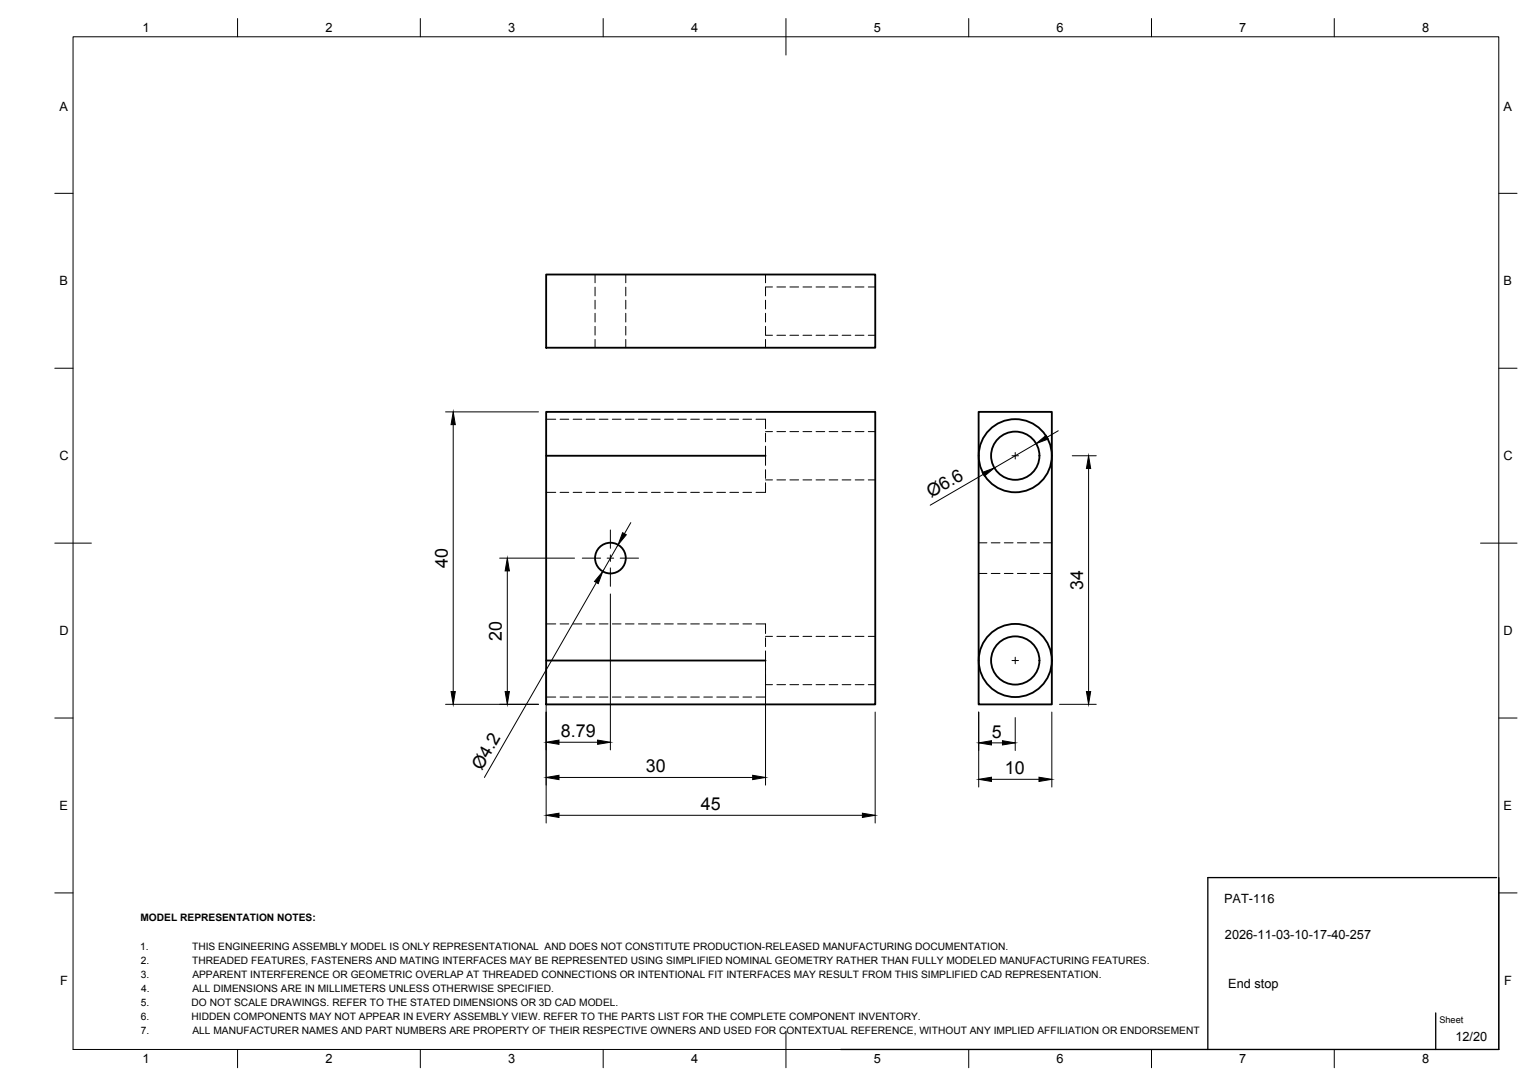
ISO-10303-21;
HEADER;
/* Generated by software containing ST-Developer
 * from STEP Tools, Inc. (www.steptools.com) 
 */

FILE_DESCRIPTION(
/* description */ ('V-block with clamp strap'),
/* implementation_level */ '2;1');

FILE_NAME(
/* name */ 'End stop.step',
/* time_stamp */ '2026-10-27T10:50:53-07:00',
/* author */ (''),
/* organization */ (''),
/* preprocessor_version */ 'ST-DEVELOPER v20.2',
/* originating_system */ 'Autodesk Translation Framework v15.17.0.0',
/* authorisation */ '');

FILE_SCHEMA (('AUTOMOTIVE_DESIGN { 1 0 10303 214 3 1 1 }'));
ENDSEC;

DATA;
#10=MECHANICAL_DESIGN_GEOMETRIC_PRESENTATION_REPRESENTATION('',(#273),#7344);
#231=SHAPE_REPRESENTATION_RELATIONSHIP('SRR','None',#7449,#252);
#252=ADVANCED_BREP_SHAPE_REPRESENTATION('',(#294),#7328);
#273=STYLED_ITEM('',(#7624),#294);
#294=MANIFOLD_SOLID_BREP('Body1',#4155);
#349=FACE_BOUND('',#954,.T.);
#350=FACE_BOUND('',#958,.T.);
#351=FACE_BOUND('',#966,.T.);
#352=FACE_BOUND('',#969,.T.);
#353=FACE_BOUND('',#971,.T.);
#354=FACE_BOUND('',#972,.T.);
#432=CIRCLE('',#4579,0.21);
#433=CIRCLE('',#4580,0.21);
#434=CIRCLE('',#4582,0.5);
#435=CIRCLE('',#4583,0.5);
#436=CIRCLE('',#4585,0.5);
#437=CIRCLE('',#4586,0.5);
#438=CIRCLE('',#4588,0.33);
#439=CIRCLE('',#4590,0.5);
#440=CIRCLE('',#4591,0.5);
#441=CIRCLE('',#4593,0.5);
#442=CIRCLE('',#4594,0.5);
#443=CIRCLE('',#4596,0.33);
#444=CIRCLE('',#4601,0.33);
#445=CIRCLE('',#4603,0.33);
#533=CYLINDRICAL_SURFACE('',#4578,0.21);
#534=CYLINDRICAL_SURFACE('',#4581,0.5);
#535=CYLINDRICAL_SURFACE('',#4584,0.5);
#536=CYLINDRICAL_SURFACE('',#4589,0.5);
#537=CYLINDRICAL_SURFACE('',#4592,0.5);
#538=CYLINDRICAL_SURFACE('',#4600,0.33);
#539=CYLINDRICAL_SURFACE('',#4602,0.33);
#666=FACE_OUTER_BOUND('',#950,.T.);
#667=FACE_OUTER_BOUND('',#951,.T.);
#668=FACE_OUTER_BOUND('',#952,.T.);
#669=FACE_OUTER_BOUND('',#953,.T.);
#670=FACE_OUTER_BOUND('',#955,.T.);
#671=FACE_OUTER_BOUND('',#956,.T.);
#672=FACE_OUTER_BOUND('',#957,.T.);
#673=FACE_OUTER_BOUND('',#959,.T.);
#674=FACE_OUTER_BOUND('',#960,.T.);
#675=FACE_OUTER_BOUND('',#961,.T.);
#676=FACE_OUTER_BOUND('',#962,.T.);
#677=FACE_OUTER_BOUND('',#963,.T.);
#678=FACE_OUTER_BOUND('',#964,.T.);
#679=FACE_OUTER_BOUND('',#965,.T.);
#680=FACE_OUTER_BOUND('',#967,.T.);
#681=FACE_OUTER_BOUND('',#968,.T.);
#682=FACE_OUTER_BOUND('',#970,.T.);
#950=EDGE_LOOP('',(#3196,#3197,#3198,#3199));
#951=EDGE_LOOP('',(#3200,#3201,#3202,#3203));
#952=EDGE_LOOP('',(#3204,#3205,#3206,#3207));
#953=EDGE_LOOP('',(#3208,#3209));
#954=EDGE_LOOP('',(#3210));
#955=EDGE_LOOP('',(#3211,#3212,#3213,#3214));
#956=EDGE_LOOP('',(#3215,#3216,#3217,#3218));
#957=EDGE_LOOP('',(#3219,#3220));
#958=EDGE_LOOP('',(#3221));
#959=EDGE_LOOP('',(#3222,#3223,#3224,#3225));
#960=EDGE_LOOP('',(#3226,#3227,#3228,#3229));
#961=EDGE_LOOP('',(#3230,#3231,#3232,#3233));
#962=EDGE_LOOP('',(#3234,#3235,#3236,#3237));
#963=EDGE_LOOP('',(#3238,#3239,#3240,#3241));
#964=EDGE_LOOP('',(#3242,#3243,#3244,#3245));
#965=EDGE_LOOP('',(#3246,#3247,#3248,#3249,#3250,#3251,#3252,#3253,#3254,
#3255));
#966=EDGE_LOOP('',(#3256));
#967=EDGE_LOOP('',(#3257,#3258,#3259,#3260));
#968=EDGE_LOOP('',(#3261,#3262,#3263,#3264,#3265,#3266,#3267,#3268,#3269,
#3270));
#969=EDGE_LOOP('',(#3271));
#970=EDGE_LOOP('',(#3272,#3273,#3274,#3275));
#971=EDGE_LOOP('',(#3276));
#972=EDGE_LOOP('',(#3277));
#1303=LINE('',#6614,#1668);
#1304=LINE('',#6619,#1669);
#1305=LINE('',#6623,#1670);
#1306=LINE('',#6626,#1671);
#1307=LINE('',#6628,#1672);
#1308=LINE('',#6636,#1673);
#1309=LINE('',#6640,#1674);
#1310=LINE('',#6643,#1675);
#1311=LINE('',#6645,#1676);
#1312=LINE('',#6652,#1677);
#1313=LINE('',#6654,#1678);
#1314=LINE('',#6655,#1679);
#1315=LINE('',#6657,#1680);
#1316=LINE('',#6658,#1681);
#1317=LINE('',#6661,#1682);
#1318=LINE('',#6663,#1683);
#1319=LINE('',#6664,#1684);
#1320=LINE('',#6668,#1685);
#1321=LINE('',#6672,#1686);
#1322=LINE('',#6676,#1687);
#1323=LINE('',#6677,#1688);
#1324=LINE('',#6678,#1689);
#1325=LINE('',#6681,#1690);
#1326=LINE('',#6682,#1691);
#1327=LINE('',#6685,#1692);
#1328=LINE('',#6686,#1693);
#1329=LINE('',#6688,#1694);
#1668=VECTOR('',#5385,0.21);
#1669=VECTOR('',#5390,1.);
#1670=VECTOR('',#5393,1.);
#1671=VECTOR('',#5398,1.);
#1672=VECTOR('',#5401,1.);
#1673=VECTOR('',#5410,1.);
#1674=VECTOR('',#5413,1.);
#1675=VECTOR('',#5418,1.);
#1676=VECTOR('',#5421,1.);
#1677=VECTOR('',#5430,1.);
#1678=VECTOR('',#5431,1.);
#1679=VECTOR('',#5432,1.);
#1680=VECTOR('',#5435,1.);
#1681=VECTOR('',#5436,1.);
#1682=VECTOR('',#5439,1.);
#1683=VECTOR('',#5440,1.);
#1684=VECTOR('',#5441,1.);
#1685=VECTOR('',#5446,0.33);
#1686=VECTOR('',#5451,0.33);
#1687=VECTOR('',#5454,1.);
#1688=VECTOR('',#5455,1.);
#1689=VECTOR('',#5456,1.);
#1690=VECTOR('',#5459,1.);
#1691=VECTOR('',#5460,1.);
#1692=VECTOR('',#5463,1.);
#1693=VECTOR('',#5464,1.);
#1694=VECTOR('',#5467,1.);
#2003=VERTEX_POINT('',#6611);
#2004=VERTEX_POINT('',#6613);
#2005=VERTEX_POINT('',#6617);
#2006=VERTEX_POINT('',#6618);
#2007=VERTEX_POINT('',#6620);
#2008=VERTEX_POINT('',#6622);
#2009=VERTEX_POINT('',#6631);
#2010=VERTEX_POINT('',#6634);
#2011=VERTEX_POINT('',#6635);
#2012=VERTEX_POINT('',#6637);
#2013=VERTEX_POINT('',#6639);
#2014=VERTEX_POINT('',#6648);
#2015=VERTEX_POINT('',#6651);
#2016=VERTEX_POINT('',#6653);
#2017=VERTEX_POINT('',#6660);
#2018=VERTEX_POINT('',#6662);
#2019=VERTEX_POINT('',#6666);
#2020=VERTEX_POINT('',#6670);
#2021=VERTEX_POINT('',#6674);
#2022=VERTEX_POINT('',#6675);
#2023=VERTEX_POINT('',#6680);
#2024=VERTEX_POINT('',#6684);
#2424=EDGE_CURVE('',#2003,#2003,#432,.T.);
#2425=EDGE_CURVE('',#2003,#2004,#1303,.T.);
#2426=EDGE_CURVE('',#2004,#2004,#433,.T.);
#2427=EDGE_CURVE('',#2005,#2006,#1304,.T.);
#2428=EDGE_CURVE('',#2007,#2006,#434,.T.);
#2429=EDGE_CURVE('',#2008,#2007,#1305,.T.);
#2430=EDGE_CURVE('',#2005,#2008,#435,.T.);
#2431=EDGE_CURVE('',#2005,#2006,#1306,.T.);
#2432=EDGE_CURVE('',#2008,#2005,#436,.T.);
#2433=EDGE_CURVE('',#2008,#2007,#1307,.T.);
#2434=EDGE_CURVE('',#2006,#2007,#437,.T.);
#2435=EDGE_CURVE('',#2009,#2009,#438,.T.);
#2436=EDGE_CURVE('',#2010,#2011,#1308,.T.);
#2437=EDGE_CURVE('',#2012,#2011,#439,.T.);
#2438=EDGE_CURVE('',#2013,#2012,#1309,.T.);
#2439=EDGE_CURVE('',#2010,#2013,#440,.T.);
#2440=EDGE_CURVE('',#2010,#2011,#1310,.T.);
#2441=EDGE_CURVE('',#2013,#2010,#441,.T.);
#2442=EDGE_CURVE('',#2013,#2012,#1311,.T.);
#2443=EDGE_CURVE('',#2011,#2012,#442,.T.);
#2444=EDGE_CURVE('',#2014,#2014,#443,.T.);
#2445=EDGE_CURVE('',#2011,#2015,#1312,.T.);
#2446=EDGE_CURVE('',#2015,#2016,#1313,.T.);
#2447=EDGE_CURVE('',#2016,#2012,#1314,.T.);
#2448=EDGE_CURVE('',#2006,#2011,#1315,.T.);
#2449=EDGE_CURVE('',#2012,#2007,#1316,.T.);
#2450=EDGE_CURVE('',#2007,#2017,#1317,.T.);
#2451=EDGE_CURVE('',#2017,#2018,#1318,.T.);
#2452=EDGE_CURVE('',#2018,#2006,#1319,.T.);
#2453=EDGE_CURVE('',#2019,#2019,#444,.T.);
#2454=EDGE_CURVE('',#2019,#2009,#1320,.T.);
#2455=EDGE_CURVE('',#2020,#2020,#445,.T.);
#2456=EDGE_CURVE('',#2020,#2014,#1321,.T.);
#2457=EDGE_CURVE('',#2021,#2022,#1322,.T.);
#2458=EDGE_CURVE('',#2022,#2016,#1323,.T.);
#2459=EDGE_CURVE('',#2021,#2015,#1324,.T.);
#2460=EDGE_CURVE('',#2023,#2021,#1325,.T.);
#2461=EDGE_CURVE('',#2023,#2018,#1326,.T.);
#2462=EDGE_CURVE('',#2024,#2023,#1327,.T.);
#2463=EDGE_CURVE('',#2024,#2017,#1328,.T.);
#2464=EDGE_CURVE('',#2022,#2024,#1329,.T.);
#3196=ORIENTED_EDGE('',*,*,#2424,.F.);
#3197=ORIENTED_EDGE('',*,*,#2425,.T.);
#3198=ORIENTED_EDGE('',*,*,#2426,.F.);
#3199=ORIENTED_EDGE('',*,*,#2425,.F.);
#3200=ORIENTED_EDGE('',*,*,#2427,.T.);
#3201=ORIENTED_EDGE('',*,*,#2428,.F.);
#3202=ORIENTED_EDGE('',*,*,#2429,.F.);
#3203=ORIENTED_EDGE('',*,*,#2430,.F.);
#3204=ORIENTED_EDGE('',*,*,#2431,.F.);
#3205=ORIENTED_EDGE('',*,*,#2432,.F.);
#3206=ORIENTED_EDGE('',*,*,#2433,.T.);
#3207=ORIENTED_EDGE('',*,*,#2434,.F.);
#3208=ORIENTED_EDGE('',*,*,#2432,.T.);
#3209=ORIENTED_EDGE('',*,*,#2430,.T.);
#3210=ORIENTED_EDGE('',*,*,#2435,.F.);
#3211=ORIENTED_EDGE('',*,*,#2436,.T.);
#3212=ORIENTED_EDGE('',*,*,#2437,.F.);
#3213=ORIENTED_EDGE('',*,*,#2438,.F.);
#3214=ORIENTED_EDGE('',*,*,#2439,.F.);
#3215=ORIENTED_EDGE('',*,*,#2440,.F.);
#3216=ORIENTED_EDGE('',*,*,#2441,.F.);
#3217=ORIENTED_EDGE('',*,*,#2442,.T.);
#3218=ORIENTED_EDGE('',*,*,#2443,.F.);
#3219=ORIENTED_EDGE('',*,*,#2441,.T.);
#3220=ORIENTED_EDGE('',*,*,#2439,.T.);
#3221=ORIENTED_EDGE('',*,*,#2444,.F.);
#3222=ORIENTED_EDGE('',*,*,#2437,.T.);
#3223=ORIENTED_EDGE('',*,*,#2445,.T.);
#3224=ORIENTED_EDGE('',*,*,#2446,.T.);
#3225=ORIENTED_EDGE('',*,*,#2447,.T.);
#3226=ORIENTED_EDGE('',*,*,#2428,.T.);
#3227=ORIENTED_EDGE('',*,*,#2448,.T.);
#3228=ORIENTED_EDGE('',*,*,#2443,.T.);
#3229=ORIENTED_EDGE('',*,*,#2449,.T.);
#3230=ORIENTED_EDGE('',*,*,#2434,.T.);
#3231=ORIENTED_EDGE('',*,*,#2450,.T.);
#3232=ORIENTED_EDGE('',*,*,#2451,.T.);
#3233=ORIENTED_EDGE('',*,*,#2452,.T.);
#3234=ORIENTED_EDGE('',*,*,#2453,.F.);
#3235=ORIENTED_EDGE('',*,*,#2454,.T.);
#3236=ORIENTED_EDGE('',*,*,#2435,.T.);
#3237=ORIENTED_EDGE('',*,*,#2454,.F.);
#3238=ORIENTED_EDGE('',*,*,#2455,.F.);
#3239=ORIENTED_EDGE('',*,*,#2456,.T.);
#3240=ORIENTED_EDGE('',*,*,#2444,.T.);
#3241=ORIENTED_EDGE('',*,*,#2456,.F.);
#3242=ORIENTED_EDGE('',*,*,#2457,.T.);
#3243=ORIENTED_EDGE('',*,*,#2458,.T.);
#3244=ORIENTED_EDGE('',*,*,#2446,.F.);
#3245=ORIENTED_EDGE('',*,*,#2459,.F.);
#3246=ORIENTED_EDGE('',*,*,#2460,.T.);
#3247=ORIENTED_EDGE('',*,*,#2459,.T.);
#3248=ORIENTED_EDGE('',*,*,#2445,.F.);
#3249=ORIENTED_EDGE('',*,*,#2436,.F.);
#3250=ORIENTED_EDGE('',*,*,#2440,.T.);
#3251=ORIENTED_EDGE('',*,*,#2448,.F.);
#3252=ORIENTED_EDGE('',*,*,#2427,.F.);
#3253=ORIENTED_EDGE('',*,*,#2431,.T.);
#3254=ORIENTED_EDGE('',*,*,#2452,.F.);
#3255=ORIENTED_EDGE('',*,*,#2461,.F.);
#3256=ORIENTED_EDGE('',*,*,#2426,.T.);
#3257=ORIENTED_EDGE('',*,*,#2462,.T.);
#3258=ORIENTED_EDGE('',*,*,#2461,.T.);
#3259=ORIENTED_EDGE('',*,*,#2451,.F.);
#3260=ORIENTED_EDGE('',*,*,#2463,.F.);
#3261=ORIENTED_EDGE('',*,*,#2464,.T.);
#3262=ORIENTED_EDGE('',*,*,#2463,.T.);
#3263=ORIENTED_EDGE('',*,*,#2450,.F.);
#3264=ORIENTED_EDGE('',*,*,#2433,.F.);
#3265=ORIENTED_EDGE('',*,*,#2429,.T.);
#3266=ORIENTED_EDGE('',*,*,#2449,.F.);
#3267=ORIENTED_EDGE('',*,*,#2442,.F.);
#3268=ORIENTED_EDGE('',*,*,#2438,.T.);
#3269=ORIENTED_EDGE('',*,*,#2447,.F.);
#3270=ORIENTED_EDGE('',*,*,#2458,.F.);
#3271=ORIENTED_EDGE('',*,*,#2424,.T.);
#3272=ORIENTED_EDGE('',*,*,#2464,.F.);
#3273=ORIENTED_EDGE('',*,*,#2457,.F.);
#3274=ORIENTED_EDGE('',*,*,#2460,.F.);
#3275=ORIENTED_EDGE('',*,*,#2462,.F.);
#3276=ORIENTED_EDGE('',*,*,#2453,.T.);
#3277=ORIENTED_EDGE('',*,*,#2455,.T.);
#3816=PLANE('',#4587);
#3817=PLANE('',#4595);
#3818=PLANE('',#4597);
#3819=PLANE('',#4598);
#3820=PLANE('',#4599);
#3821=PLANE('',#4604);
#3822=PLANE('',#4605);
#3823=PLANE('',#4606);
#3824=PLANE('',#4607);
#3825=PLANE('',#4608);
#4012=ADVANCED_FACE('',(#666),#533,.F.);
#4013=ADVANCED_FACE('',(#667),#534,.F.);
#4014=ADVANCED_FACE('',(#668),#535,.F.);
#4015=ADVANCED_FACE('',(#669,#349),#3816,.T.);
#4016=ADVANCED_FACE('',(#670),#536,.F.);
#4017=ADVANCED_FACE('',(#671),#537,.F.);
#4018=ADVANCED_FACE('',(#672,#350),#3817,.T.);
#4019=ADVANCED_FACE('',(#673),#3818,.T.);
#4020=ADVANCED_FACE('',(#674),#3819,.T.);
#4021=ADVANCED_FACE('',(#675),#3820,.T.);
#4022=ADVANCED_FACE('',(#676),#538,.F.);
#4023=ADVANCED_FACE('',(#677),#539,.F.);
#4024=ADVANCED_FACE('',(#678),#3821,.T.);
#4025=ADVANCED_FACE('',(#679,#351),#3822,.T.);
#4026=ADVANCED_FACE('',(#680),#3823,.T.);
#4027=ADVANCED_FACE('',(#681,#352),#3824,.T.);
#4028=ADVANCED_FACE('',(#682,#353,#354),#3825,.F.);
#4155=CLOSED_SHELL('',(#4012,#4013,#4014,#4015,#4016,#4017,#4018,#4019,
#4020,#4021,#4022,#4023,#4024,#4025,#4026,#4027,#4028));
#4577=AXIS2_PLACEMENT_3D('',#6609,#5379,#5380);
#4578=AXIS2_PLACEMENT_3D('',#6610,#5381,#5382);
#4579=AXIS2_PLACEMENT_3D('',#6612,#5383,#5384);
#4580=AXIS2_PLACEMENT_3D('',#6615,#5386,#5387);
#4581=AXIS2_PLACEMENT_3D('',#6616,#5388,#5389);
#4582=AXIS2_PLACEMENT_3D('',#6621,#5391,#5392);
#4583=AXIS2_PLACEMENT_3D('',#6624,#5394,#5395);
#4584=AXIS2_PLACEMENT_3D('',#6625,#5396,#5397);
#4585=AXIS2_PLACEMENT_3D('',#6627,#5399,#5400);
#4586=AXIS2_PLACEMENT_3D('',#6629,#5402,#5403);
#4587=AXIS2_PLACEMENT_3D('',#6630,#5404,#5405);
#4588=AXIS2_PLACEMENT_3D('',#6632,#5406,#5407);
#4589=AXIS2_PLACEMENT_3D('',#6633,#5408,#5409);
#4590=AXIS2_PLACEMENT_3D('',#6638,#5411,#5412);
#4591=AXIS2_PLACEMENT_3D('',#6641,#5414,#5415);
#4592=AXIS2_PLACEMENT_3D('',#6642,#5416,#5417);
#4593=AXIS2_PLACEMENT_3D('',#6644,#5419,#5420);
#4594=AXIS2_PLACEMENT_3D('',#6646,#5422,#5423);
#4595=AXIS2_PLACEMENT_3D('',#6647,#5424,#5425);
#4596=AXIS2_PLACEMENT_3D('',#6649,#5426,#5427);
#4597=AXIS2_PLACEMENT_3D('',#6650,#5428,#5429);
#4598=AXIS2_PLACEMENT_3D('',#6656,#5433,#5434);
#4599=AXIS2_PLACEMENT_3D('',#6659,#5437,#5438);
#4600=AXIS2_PLACEMENT_3D('',#6665,#5442,#5443);
#4601=AXIS2_PLACEMENT_3D('',#6667,#5444,#5445);
#4602=AXIS2_PLACEMENT_3D('',#6669,#5447,#5448);
#4603=AXIS2_PLACEMENT_3D('',#6671,#5449,#5450);
#4604=AXIS2_PLACEMENT_3D('',#6673,#5452,#5453);
#4605=AXIS2_PLACEMENT_3D('',#6679,#5457,#5458);
#4606=AXIS2_PLACEMENT_3D('',#6683,#5461,#5462);
#4607=AXIS2_PLACEMENT_3D('',#6687,#5465,#5466);
#4608=AXIS2_PLACEMENT_3D('',#6689,#5468,#5469);
#5379=DIRECTION('axis',(0.,0.,1.));
#5380=DIRECTION('refdir',(1.,0.,0.));
#5381=DIRECTION('center_axis',(1.,0.,0.));
#5382=DIRECTION('ref_axis',(0.,0.,-1.));
#5383=DIRECTION('center_axis',(1.,0.,0.));
#5384=DIRECTION('ref_axis',(0.,0.,-1.));
#5385=DIRECTION('',(1.,0.,0.));
#5386=DIRECTION('center_axis',(-1.,0.,0.));
#5387=DIRECTION('ref_axis',(0.,0.,-1.));
#5388=DIRECTION('center_axis',(0.,0.,1.));
#5389=DIRECTION('ref_axis',(1.,0.,0.));
#5390=DIRECTION('',(0.,0.,1.));
#5391=DIRECTION('center_axis',(0.,0.,-1.));
#5392=DIRECTION('ref_axis',(1.,0.,0.));
#5393=DIRECTION('',(0.,0.,1.));
#5394=DIRECTION('center_axis',(0.,0.,1.));
#5395=DIRECTION('ref_axis',(1.,0.,0.));
#5396=DIRECTION('center_axis',(0.,0.,1.));
#5397=DIRECTION('ref_axis',(1.,0.,0.));
#5398=DIRECTION('',(0.,0.,1.));
#5399=DIRECTION('center_axis',(0.,0.,1.));
#5400=DIRECTION('ref_axis',(1.,0.,0.));
#5401=DIRECTION('',(0.,0.,1.));
#5402=DIRECTION('center_axis',(0.,0.,-1.));
#5403=DIRECTION('ref_axis',(1.,0.,0.));
#5404=DIRECTION('center_axis',(0.,0.,1.));
#5405=DIRECTION('ref_axis',(1.,0.,0.));
#5406=DIRECTION('center_axis',(0.,0.,1.));
#5407=DIRECTION('ref_axis',(1.,0.,0.));
#5408=DIRECTION('center_axis',(0.,0.,1.));
#5409=DIRECTION('ref_axis',(1.,0.,0.));
#5410=DIRECTION('',(0.,0.,1.));
#5411=DIRECTION('center_axis',(0.,0.,-1.));
#5412=DIRECTION('ref_axis',(1.,0.,0.));
#5413=DIRECTION('',(0.,0.,1.));
#5414=DIRECTION('center_axis',(0.,0.,1.));
#5415=DIRECTION('ref_axis',(1.,0.,0.));
#5416=DIRECTION('center_axis',(0.,0.,1.));
#5417=DIRECTION('ref_axis',(1.,0.,0.));
#5418=DIRECTION('',(0.,0.,1.));
#5419=DIRECTION('center_axis',(0.,0.,1.));
#5420=DIRECTION('ref_axis',(1.,0.,0.));
#5421=DIRECTION('',(0.,0.,1.));
#5422=DIRECTION('center_axis',(0.,0.,-1.));
#5423=DIRECTION('ref_axis',(1.,0.,0.));
#5424=DIRECTION('center_axis',(0.,0.,1.));
#5425=DIRECTION('ref_axis',(1.,0.,0.));
#5426=DIRECTION('center_axis',(0.,0.,1.));
#5427=DIRECTION('ref_axis',(1.,0.,0.));
#5428=DIRECTION('center_axis',(0.,0.,1.));
#5429=DIRECTION('ref_axis',(1.,0.,0.));
#5430=DIRECTION('',(0.,1.,0.));
#5431=DIRECTION('',(-1.,0.,0.));
#5432=DIRECTION('',(0.,-1.,0.));
#5433=DIRECTION('center_axis',(0.,0.,1.));
#5434=DIRECTION('ref_axis',(1.,0.,0.));
#5435=DIRECTION('',(0.,1.,0.));
#5436=DIRECTION('',(0.,-1.,0.));
#5437=DIRECTION('center_axis',(0.,0.,1.));
#5438=DIRECTION('ref_axis',(1.,0.,0.));
#5439=DIRECTION('',(0.,-1.,0.));
#5440=DIRECTION('',(1.,0.,0.));
#5441=DIRECTION('',(0.,1.,0.));
#5442=DIRECTION('center_axis',(0.,0.,1.));
#5443=DIRECTION('ref_axis',(1.,0.,0.));
#5444=DIRECTION('center_axis',(0.,0.,1.));
#5445=DIRECTION('ref_axis',(1.,0.,0.));
#5446=DIRECTION('',(0.,0.,1.));
#5447=DIRECTION('center_axis',(0.,0.,1.));
#5448=DIRECTION('ref_axis',(1.,0.,0.));
#5449=DIRECTION('center_axis',(0.,0.,1.));
#5450=DIRECTION('ref_axis',(1.,0.,0.));
#5451=DIRECTION('',(0.,0.,1.));
#5452=DIRECTION('center_axis',(0.,1.,0.));
#5453=DIRECTION('ref_axis',(-1.,0.,0.));
#5454=DIRECTION('',(-1.,0.,0.));
#5455=DIRECTION('',(0.,0.,1.));
#5456=DIRECTION('',(0.,0.,1.));
#5457=DIRECTION('center_axis',(1.,0.,0.));
#5458=DIRECTION('ref_axis',(0.,1.,0.));
#5459=DIRECTION('',(0.,1.,0.));
#5460=DIRECTION('',(0.,0.,1.));
#5461=DIRECTION('center_axis',(0.,-1.,0.));
#5462=DIRECTION('ref_axis',(1.,0.,0.));
#5463=DIRECTION('',(1.,0.,0.));
#5464=DIRECTION('',(0.,0.,1.));
#5465=DIRECTION('center_axis',(-1.,0.,0.));
#5466=DIRECTION('ref_axis',(0.,-1.,0.));
#5467=DIRECTION('',(0.,-1.,0.));
#5468=DIRECTION('center_axis',(0.,0.,1.));
#5469=DIRECTION('ref_axis',(1.,0.,0.));
#6609=CARTESIAN_POINT('',(0.,0.,0.));
#6610=CARTESIAN_POINT('Origin',(1.4,0.,4.62132034355964));
#6611=CARTESIAN_POINT('',(1.5,-2.57175827820944E-17,4.83132034355964));
#6612=CARTESIAN_POINT('Origin',(1.5,0.,4.62132034355964));
#6613=CARTESIAN_POINT('',(2.5,2.57175827820944E-17,4.83132034355964));
#6614=CARTESIAN_POINT('',(1.4,-2.57175827820944E-17,4.83132034355964));
#6615=CARTESIAN_POINT('Origin',(2.5,0.,4.62132034355964));
#6616=CARTESIAN_POINT('Origin',(2.,-1.4,2.5));
#6617=CARTESIAN_POINT('',(2.5,-1.4,2.5));
#6618=CARTESIAN_POINT('',(2.5,-1.4,5.5));
#6619=CARTESIAN_POINT('',(2.5,-1.4,2.5));
#6620=CARTESIAN_POINT('',(1.5,-1.4,5.5));
#6621=CARTESIAN_POINT('Origin',(2.,-1.4,5.5));
#6622=CARTESIAN_POINT('',(1.5,-1.4,2.5));
#6623=CARTESIAN_POINT('',(1.5,-1.4,2.5));
#6624=CARTESIAN_POINT('Origin',(2.,-1.4,2.5));
#6625=CARTESIAN_POINT('Origin',(2.,-1.4,2.5));
#6626=CARTESIAN_POINT('',(2.5,-1.4,2.5));
#6627=CARTESIAN_POINT('Origin',(2.,-1.4,2.5));
#6628=CARTESIAN_POINT('',(1.5,-1.4,2.5));
#6629=CARTESIAN_POINT('Origin',(2.,-1.4,5.5));
#6630=CARTESIAN_POINT('Origin',(2.,-1.4,2.5));
#6631=CARTESIAN_POINT('',(1.67,-1.4,2.5));
#6632=CARTESIAN_POINT('Origin',(2.,-1.4,2.5));
#6633=CARTESIAN_POINT('Origin',(2.,1.4,2.5));
#6634=CARTESIAN_POINT('',(2.5,1.4,2.5));
#6635=CARTESIAN_POINT('',(2.5,1.4,5.5));
#6636=CARTESIAN_POINT('',(2.5,1.4,2.5));
#6637=CARTESIAN_POINT('',(1.5,1.4,5.5));
#6638=CARTESIAN_POINT('Origin',(2.,1.4,5.5));
#6639=CARTESIAN_POINT('',(1.5,1.4,2.5));
#6640=CARTESIAN_POINT('',(1.5,1.4,2.5));
#6641=CARTESIAN_POINT('Origin',(2.,1.4,2.5));
#6642=CARTESIAN_POINT('Origin',(2.,1.4,2.5));
#6643=CARTESIAN_POINT('',(2.5,1.4,2.5));
#6644=CARTESIAN_POINT('Origin',(2.,1.4,2.5));
#6645=CARTESIAN_POINT('',(1.5,1.4,2.5));
#6646=CARTESIAN_POINT('Origin',(2.,1.4,5.5));
#6647=CARTESIAN_POINT('Origin',(2.,1.4,2.5));
#6648=CARTESIAN_POINT('',(1.67,1.4,2.5));
#6649=CARTESIAN_POINT('Origin',(2.,1.4,2.5));
#6650=CARTESIAN_POINT('Origin',(2.,0.,5.5));
#6651=CARTESIAN_POINT('',(2.5,2.,5.5));
#6652=CARTESIAN_POINT('',(2.5,-2.,5.5));
#6653=CARTESIAN_POINT('',(1.5,2.,5.5));
#6654=CARTESIAN_POINT('',(2.5,2.,5.5));
#6655=CARTESIAN_POINT('',(1.5,2.,5.5));
#6656=CARTESIAN_POINT('Origin',(2.,0.,5.5));
#6657=CARTESIAN_POINT('',(2.5,-2.,5.5));
#6658=CARTESIAN_POINT('',(1.5,2.,5.5));
#6659=CARTESIAN_POINT('Origin',(2.,0.,5.5));
#6660=CARTESIAN_POINT('',(1.5,-2.,5.5));
#6661=CARTESIAN_POINT('',(1.5,2.,5.5));
#6662=CARTESIAN_POINT('',(2.5,-2.,5.5));
#6663=CARTESIAN_POINT('',(1.5,-2.,5.5));
#6664=CARTESIAN_POINT('',(2.5,-2.,5.5));
#6665=CARTESIAN_POINT('Origin',(2.,-1.4,0.9));
#6666=CARTESIAN_POINT('',(1.67,-1.4,1.));
#6667=CARTESIAN_POINT('Origin',(2.,-1.4,1.));
#6668=CARTESIAN_POINT('',(1.67,-1.4,0.9));
#6669=CARTESIAN_POINT('Origin',(2.,1.4,0.9));
#6670=CARTESIAN_POINT('',(1.67,1.4,1.));
#6671=CARTESIAN_POINT('Origin',(2.,1.4,1.));
#6672=CARTESIAN_POINT('',(1.67,1.4,0.9));
#6673=CARTESIAN_POINT('Origin',(2.5,2.,1.));
#6674=CARTESIAN_POINT('',(2.5,2.,1.));
#6675=CARTESIAN_POINT('',(1.5,2.,1.));
#6676=CARTESIAN_POINT('',(2.5,2.,1.));
#6677=CARTESIAN_POINT('',(1.5,2.,1.));
#6678=CARTESIAN_POINT('',(2.5,2.,1.));
#6679=CARTESIAN_POINT('Origin',(2.5,-2.,1.));
#6680=CARTESIAN_POINT('',(2.5,-2.,1.));
#6681=CARTESIAN_POINT('',(2.5,-2.,1.));
#6682=CARTESIAN_POINT('',(2.5,-2.,1.));
#6683=CARTESIAN_POINT('Origin',(1.5,-2.,1.));
#6684=CARTESIAN_POINT('',(1.5,-2.,1.));
#6685=CARTESIAN_POINT('',(1.5,-2.,1.));
#6686=CARTESIAN_POINT('',(1.5,-2.,1.));
#6687=CARTESIAN_POINT('Origin',(1.5,2.,1.));
#6688=CARTESIAN_POINT('',(1.5,2.,1.));
#6689=CARTESIAN_POINT('Origin',(2.,0.,1.));
#7302=UNCERTAINTY_MEASURE_WITH_UNIT(LENGTH_MEASURE(0.001),#7345,
'DISTANCE_ACCURACY_VALUE',
'Maximum model space distance between geometric entities at asserted c
onnectivities');
#7318=UNCERTAINTY_MEASURE_WITH_UNIT(LENGTH_MEASURE(0.001),#7345,
'DISTANCE_ACCURACY_VALUE',
'Maximum model space distance between geometric entities at asserted c
onnectivities');
#7328=(
GEOMETRIC_REPRESENTATION_CONTEXT(3)
GLOBAL_UNCERTAINTY_ASSIGNED_CONTEXT((#7302))
GLOBAL_UNIT_ASSIGNED_CONTEXT((#7345,#7347,#7348))
REPRESENTATION_CONTEXT('','3D')
);
#7344=(
GEOMETRIC_REPRESENTATION_CONTEXT(3)
GLOBAL_UNCERTAINTY_ASSIGNED_CONTEXT((#7318))
GLOBAL_UNIT_ASSIGNED_CONTEXT((#7345,#7347,#7348))
REPRESENTATION_CONTEXT('','3D')
);
#7345=(
LENGTH_UNIT()
NAMED_UNIT(*)
SI_UNIT(.CENTI.,.METRE.)
);
#7347=(
NAMED_UNIT(*)
PLANE_ANGLE_UNIT()
SI_UNIT($,.RADIAN.)
);
#7348=(
NAMED_UNIT(*)
SI_UNIT($,.STERADIAN.)
SOLID_ANGLE_UNIT()
);
#7358=SHAPE_DEFINITION_REPRESENTATION(#7383,#7449);
#7383=PRODUCT_DEFINITION_SHAPE('',$,#7475);
#7449=SHAPE_REPRESENTATION('',(#4577),#7328);
#7465=PRODUCT_DEFINITION_CONTEXT('part definition',#7542,'design');
#7475=PRODUCT_DEFINITION('End stop','End stop',#7500,#7465);
#7500=PRODUCT_DEFINITION_FORMATION('',$,#7553);
#7542=APPLICATION_CONTEXT(
'Core Data for Automotive Mechanical Design Process');
#7543=PRODUCT_CONTEXT('part definition',#7542,'mechanical');
#7553=PRODUCT('End stop','End stop','End stop',(#7543));
#7618=COLOUR_RGB('Sky Blue',0.24,0.69,0.87);
#7619=FILL_AREA_STYLE_COLOUR('',#7618);
#7620=FILL_AREA_STYLE('',(#7619));
#7621=SURFACE_STYLE_FILL_AREA(#7620);
#7622=SURFACE_SIDE_STYLE('',(#7621));
#7623=SURFACE_STYLE_USAGE(.BOTH.,#7622);
#7624=PRESENTATION_STYLE_ASSIGNMENT((#7623));
ENDSEC;
END-ISO-10303-21;
